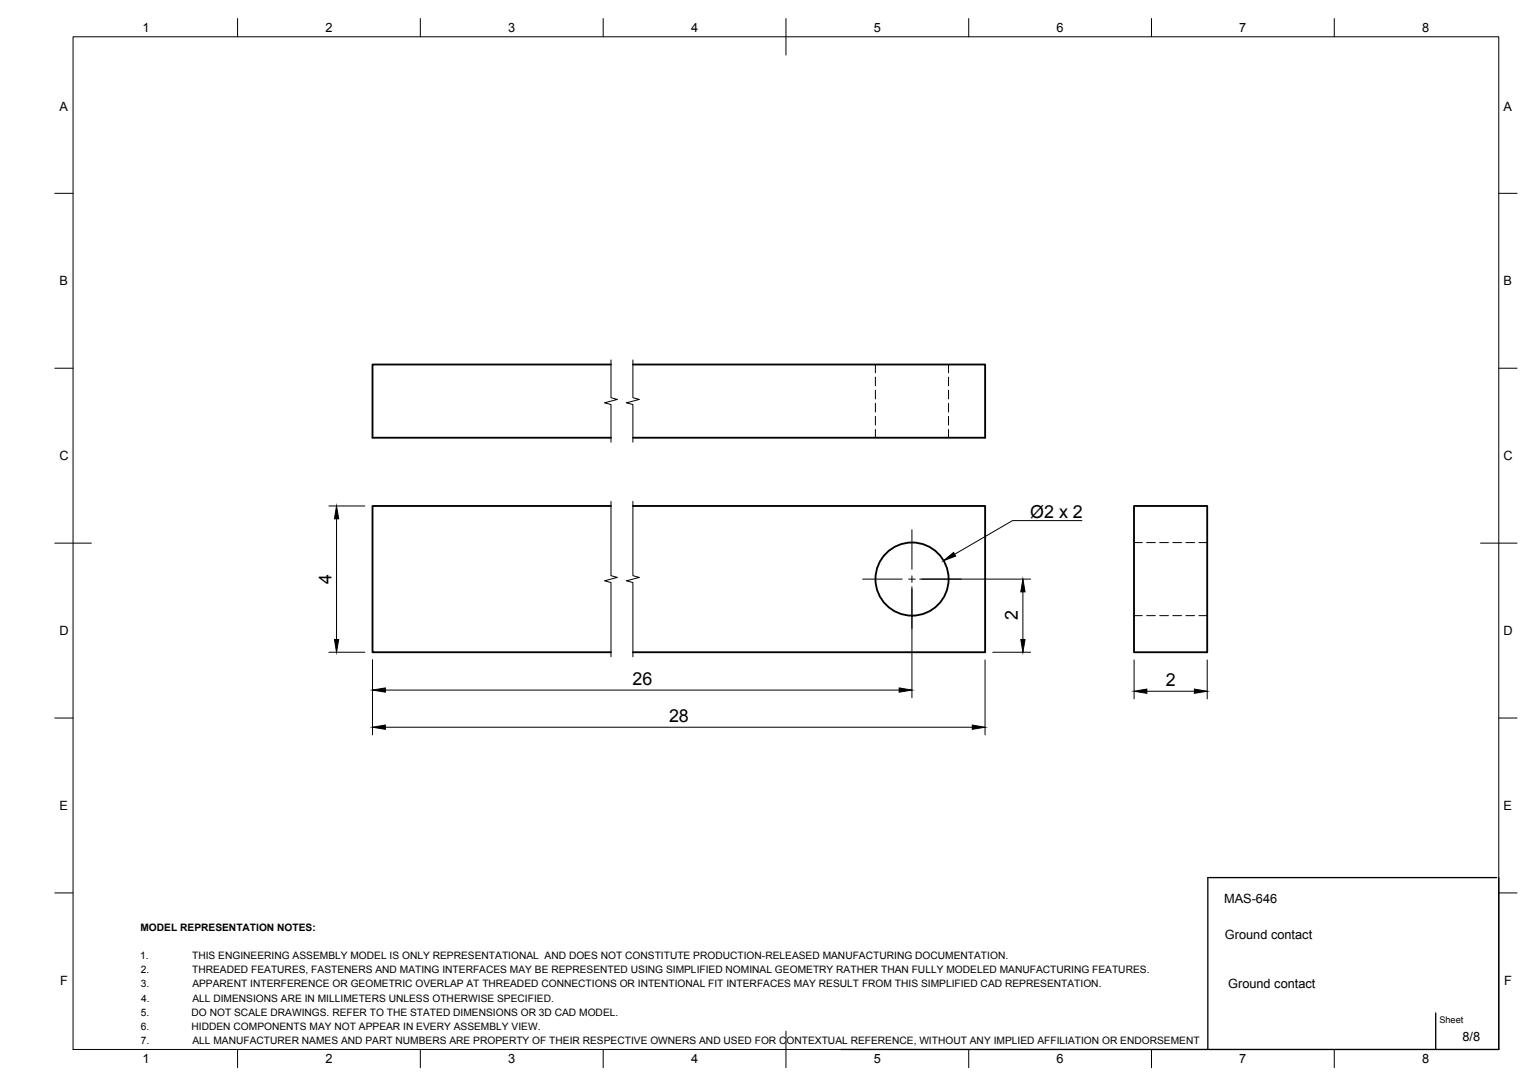
ISO-10303-21;
HEADER;
/* Generated by software containing ST-Developer
 * from STEP Tools, Inc. (www.steptools.com) 
 */

FILE_DESCRIPTION(
/* description */ ('Independent keyed three-contact power inlet for the IEC-connector des
ign category. Longer ground blade, retained contacts, wire termination
 holes and sealed bolted panel interface. Nominal custom interface; IE
C dimensional compatibility and electrical ratings are not assigned.'),

/* implementation_level */ '2;1');

FILE_NAME(
/* name */ 'Ground contact.step',
/* time_stamp */ '2026-11-08T19:55:04-08:00',
/* author */ (''),
/* organization */ (''),
/* preprocessor_version */ 'ST-DEVELOPER v20.2',
/* originating_system */ 'Autodesk Translation Framework v15.17.0.0',
/* authorisation */ '');

FILE_SCHEMA (('AUTOMOTIVE_DESIGN { 1 0 10303 214 3 1 1 }'));
ENDSEC;

DATA;
#10=MECHANICAL_DESIGN_GEOMETRIC_PRESENTATION_REPRESENTATION('',(#113),#21880);
#93=SHAPE_REPRESENTATION_RELATIONSHIP('SRR','None',#21929,#103);
#103=ADVANCED_BREP_SHAPE_REPRESENTATION('',(#123),#21874);
#113=STYLED_ITEM('',(#21988),#123);
#123=MANIFOLD_SOLID_BREP('Body1',#6385);
#185=FACE_BOUND('',#935,.T.);
#186=FACE_BOUND('',#938,.T.);
#271=PLANE('',#6806);
#272=PLANE('',#6807);
#273=PLANE('',#6808);
#274=PLANE('',#6809);
#275=PLANE('',#6810);
#276=PLANE('',#6811);
#547=FACE_OUTER_BOUND('',#933,.T.);
#548=FACE_OUTER_BOUND('',#934,.T.);
#549=FACE_OUTER_BOUND('',#936,.T.);
#550=FACE_OUTER_BOUND('',#937,.T.);
#551=FACE_OUTER_BOUND('',#939,.T.);
#552=FACE_OUTER_BOUND('',#940,.T.);
#553=FACE_OUTER_BOUND('',#941,.T.);
#933=EDGE_LOOP('',(#5195,#5196,#5197,#5198));
#934=EDGE_LOOP('',(#5199,#5200,#5201,#5202));
#935=EDGE_LOOP('',(#5203));
#936=EDGE_LOOP('',(#5204,#5205,#5206,#5207));
#937=EDGE_LOOP('',(#5208,#5209,#5210,#5211));
#938=EDGE_LOOP('',(#5212));
#939=EDGE_LOOP('',(#5213,#5214,#5215,#5216));
#940=EDGE_LOOP('',(#5217,#5218,#5219,#5220));
#941=EDGE_LOOP('',(#5221,#5222,#5223,#5224));
#1136=CIRCLE('',#6804,1.);
#1137=CIRCLE('',#6805,1.);
#1839=LINE('',#16286,#2295);
#1840=LINE('',#16291,#2296);
#1841=LINE('',#16293,#2297);
#1842=LINE('',#16295,#2298);
#1843=LINE('',#16296,#2299);
#1844=LINE('',#16299,#2300);
#1845=LINE('',#16301,#2301);
#1846=LINE('',#16302,#2302);
#1847=LINE('',#16305,#2303);
#1848=LINE('',#16307,#2304);
#1849=LINE('',#16308,#2305);
#1850=LINE('',#16310,#2306);
#1851=LINE('',#16311,#2307);
#2295=VECTOR('',#7883,1.);
#2296=VECTOR('',#7888,10.);
#2297=VECTOR('',#7889,10.);
#2298=VECTOR('',#7890,10.);
#2299=VECTOR('',#7891,10.);
#2300=VECTOR('',#7894,10.);
#2301=VECTOR('',#7895,10.);
#2302=VECTOR('',#7896,10.);
#2303=VECTOR('',#7899,10.);
#2304=VECTOR('',#7900,10.);
#2305=VECTOR('',#7901,10.);
#2306=VECTOR('',#7904,10.);
#2307=VECTOR('',#7905,10.);
#2835=VERTEX_POINT('',#16283);
#2836=VERTEX_POINT('',#16285);
#2837=VERTEX_POINT('',#16289);
#2838=VERTEX_POINT('',#16290);
#2839=VERTEX_POINT('',#16292);
#2840=VERTEX_POINT('',#16294);
#2841=VERTEX_POINT('',#16298);
#2842=VERTEX_POINT('',#16300);
#2843=VERTEX_POINT('',#16304);
#2844=VERTEX_POINT('',#16306);
#3657=EDGE_CURVE('',#2835,#2835,#1136,.T.);
#3658=EDGE_CURVE('',#2835,#2836,#1839,.T.);
#3659=EDGE_CURVE('',#2836,#2836,#1137,.T.);
#3660=EDGE_CURVE('',#2837,#2838,#1840,.T.);
#3661=EDGE_CURVE('',#2838,#2839,#1841,.T.);
#3662=EDGE_CURVE('',#2840,#2839,#1842,.T.);
#3663=EDGE_CURVE('',#2837,#2840,#1843,.T.);
#3664=EDGE_CURVE('',#2841,#2837,#1844,.T.);
#3665=EDGE_CURVE('',#2842,#2840,#1845,.T.);
#3666=EDGE_CURVE('',#2841,#2842,#1846,.T.);
#3667=EDGE_CURVE('',#2843,#2841,#1847,.T.);
#3668=EDGE_CURVE('',#2844,#2842,#1848,.T.);
#3669=EDGE_CURVE('',#2843,#2844,#1849,.T.);
#3670=EDGE_CURVE('',#2838,#2843,#1850,.T.);
#3671=EDGE_CURVE('',#2839,#2844,#1851,.T.);
#5195=ORIENTED_EDGE('',*,*,#3657,.F.);
#5196=ORIENTED_EDGE('',*,*,#3658,.T.);
#5197=ORIENTED_EDGE('',*,*,#3659,.F.);
#5198=ORIENTED_EDGE('',*,*,#3658,.F.);
#5199=ORIENTED_EDGE('',*,*,#3660,.T.);
#5200=ORIENTED_EDGE('',*,*,#3661,.T.);
#5201=ORIENTED_EDGE('',*,*,#3662,.F.);
#5202=ORIENTED_EDGE('',*,*,#3663,.F.);
#5203=ORIENTED_EDGE('',*,*,#3657,.T.);
#5204=ORIENTED_EDGE('',*,*,#3664,.T.);
#5205=ORIENTED_EDGE('',*,*,#3663,.T.);
#5206=ORIENTED_EDGE('',*,*,#3665,.F.);
#5207=ORIENTED_EDGE('',*,*,#3666,.F.);
#5208=ORIENTED_EDGE('',*,*,#3667,.T.);
#5209=ORIENTED_EDGE('',*,*,#3666,.T.);
#5210=ORIENTED_EDGE('',*,*,#3668,.F.);
#5211=ORIENTED_EDGE('',*,*,#3669,.F.);
#5212=ORIENTED_EDGE('',*,*,#3659,.T.);
#5213=ORIENTED_EDGE('',*,*,#3670,.T.);
#5214=ORIENTED_EDGE('',*,*,#3669,.T.);
#5215=ORIENTED_EDGE('',*,*,#3671,.F.);
#5216=ORIENTED_EDGE('',*,*,#3661,.F.);
#5217=ORIENTED_EDGE('',*,*,#3671,.T.);
#5218=ORIENTED_EDGE('',*,*,#3668,.T.);
#5219=ORIENTED_EDGE('',*,*,#3665,.T.);
#5220=ORIENTED_EDGE('',*,*,#3662,.T.);
#5221=ORIENTED_EDGE('',*,*,#3670,.F.);
#5222=ORIENTED_EDGE('',*,*,#3660,.F.);
#5223=ORIENTED_EDGE('',*,*,#3664,.F.);
#5224=ORIENTED_EDGE('',*,*,#3667,.F.);
#5963=CYLINDRICAL_SURFACE('',#6803,1.);
#6259=ADVANCED_FACE('',(#547),#5963,.F.);
#6260=ADVANCED_FACE('',(#548,#185),#271,.T.);
#6261=ADVANCED_FACE('',(#549),#272,.T.);
#6262=ADVANCED_FACE('',(#550,#186),#273,.T.);
#6263=ADVANCED_FACE('',(#551),#274,.T.);
#6264=ADVANCED_FACE('',(#552),#275,.T.);
#6265=ADVANCED_FACE('',(#553),#276,.F.);
#6385=CLOSED_SHELL('',(#6259,#6260,#6261,#6262,#6263,#6264,#6265));
#6802=AXIS2_PLACEMENT_3D('',#16281,#7877,#7878);
#6803=AXIS2_PLACEMENT_3D('',#16282,#7879,#7880);
#6804=AXIS2_PLACEMENT_3D('',#16284,#7881,#7882);
#6805=AXIS2_PLACEMENT_3D('',#16287,#7884,#7885);
#6806=AXIS2_PLACEMENT_3D('',#16288,#7886,#7887);
#6807=AXIS2_PLACEMENT_3D('',#16297,#7892,#7893);
#6808=AXIS2_PLACEMENT_3D('',#16303,#7897,#7898);
#6809=AXIS2_PLACEMENT_3D('',#16309,#7902,#7903);
#6810=AXIS2_PLACEMENT_3D('',#16312,#7906,#7907);
#6811=AXIS2_PLACEMENT_3D('',#16313,#7908,#7909);
#7877=DIRECTION('axis',(0.,0.,1.));
#7878=DIRECTION('refdir',(1.,0.,0.));
#7879=DIRECTION('center_axis',(0.,-1.,0.));
#7880=DIRECTION('ref_axis',(0.,0.,1.));
#7881=DIRECTION('center_axis',(0.,-1.,0.));
#7882=DIRECTION('ref_axis',(0.,0.,1.));
#7883=DIRECTION('',(0.,-1.,0.));
#7884=DIRECTION('center_axis',(0.,1.,0.));
#7885=DIRECTION('ref_axis',(0.,0.,1.));
#7886=DIRECTION('center_axis',(0.,1.,0.));
#7887=DIRECTION('ref_axis',(-1.,0.,0.));
#7888=DIRECTION('',(-1.,0.,0.));
#7889=DIRECTION('',(0.,0.,1.));
#7890=DIRECTION('',(-1.,0.,0.));
#7891=DIRECTION('',(0.,0.,1.));
#7892=DIRECTION('center_axis',(1.,0.,0.));
#7893=DIRECTION('ref_axis',(0.,1.,0.));
#7894=DIRECTION('',(0.,1.,0.));
#7895=DIRECTION('',(0.,1.,0.));
#7896=DIRECTION('',(0.,0.,1.));
#7897=DIRECTION('center_axis',(0.,-1.,0.));
#7898=DIRECTION('ref_axis',(1.,0.,0.));
#7899=DIRECTION('',(1.,0.,0.));
#7900=DIRECTION('',(1.,0.,0.));
#7901=DIRECTION('',(0.,0.,1.));
#7902=DIRECTION('center_axis',(-1.,0.,0.));
#7903=DIRECTION('ref_axis',(0.,-1.,0.));
#7904=DIRECTION('',(0.,-1.,0.));
#7905=DIRECTION('',(0.,-1.,0.));
#7906=DIRECTION('center_axis',(0.,0.,1.));
#7907=DIRECTION('ref_axis',(1.,0.,0.));
#7908=DIRECTION('center_axis',(0.,0.,1.));
#7909=DIRECTION('ref_axis',(1.,0.,0.));
#16281=CARTESIAN_POINT('',(0.,0.,0.));
#16282=CARTESIAN_POINT('Origin',(0.,0.,2.));
#16283=CARTESIAN_POINT('',(1.22464679914735E-16,1.,1.));
#16284=CARTESIAN_POINT('Origin',(0.,1.,2.));
#16285=CARTESIAN_POINT('',(1.22464679914735E-16,-1.,1.));
#16286=CARTESIAN_POINT('',(1.22464679914735E-16,0.,1.));
#16287=CARTESIAN_POINT('Origin',(0.,-1.,2.));
#16288=CARTESIAN_POINT('Origin',(2.,1.,0.));
#16289=CARTESIAN_POINT('',(2.,1.,0.));
#16290=CARTESIAN_POINT('',(-2.,1.,0.));
#16291=CARTESIAN_POINT('',(2.,1.,0.));
#16292=CARTESIAN_POINT('',(-2.,1.,28.));
#16293=CARTESIAN_POINT('',(-2.,1.,0.));
#16294=CARTESIAN_POINT('',(2.,1.,28.));
#16295=CARTESIAN_POINT('',(2.,1.,28.));
#16296=CARTESIAN_POINT('',(2.,1.,0.));
#16297=CARTESIAN_POINT('Origin',(2.,-1.,0.));
#16298=CARTESIAN_POINT('',(2.,-1.,0.));
#16299=CARTESIAN_POINT('',(2.,-1.,0.));
#16300=CARTESIAN_POINT('',(2.,-1.,28.));
#16301=CARTESIAN_POINT('',(2.,-1.,28.));
#16302=CARTESIAN_POINT('',(2.,-1.,0.));
#16303=CARTESIAN_POINT('Origin',(-2.,-1.,0.));
#16304=CARTESIAN_POINT('',(-2.,-1.,0.));
#16305=CARTESIAN_POINT('',(-2.,-1.,0.));
#16306=CARTESIAN_POINT('',(-2.,-1.,28.));
#16307=CARTESIAN_POINT('',(-2.,-1.,28.));
#16308=CARTESIAN_POINT('',(-2.,-1.,0.));
#16309=CARTESIAN_POINT('Origin',(-2.,1.,0.));
#16310=CARTESIAN_POINT('',(-2.,1.,0.));
#16311=CARTESIAN_POINT('',(-2.,1.,28.));
#16312=CARTESIAN_POINT('Origin',(0.,0.,28.));
#16313=CARTESIAN_POINT('Origin',(0.,0.,0.));
#21862=UNCERTAINTY_MEASURE_WITH_UNIT(LENGTH_MEASURE(0.01),#21881,
'DISTANCE_ACCURACY_VALUE',
'Maximum model space distance between geometric entities at asserted c
onnectivities');
#21868=UNCERTAINTY_MEASURE_WITH_UNIT(LENGTH_MEASURE(0.01),#21881,
'DISTANCE_ACCURACY_VALUE',
'Maximum model space distance between geometric entities at asserted c
onnectivities');
#21874=(
GEOMETRIC_REPRESENTATION_CONTEXT(3)
GLOBAL_UNCERTAINTY_ASSIGNED_CONTEXT((#21862))
GLOBAL_UNIT_ASSIGNED_CONTEXT((#21881,#21883,#21884))
REPRESENTATION_CONTEXT('','3D')
);
#21880=(
GEOMETRIC_REPRESENTATION_CONTEXT(3)
GLOBAL_UNCERTAINTY_ASSIGNED_CONTEXT((#21868))
GLOBAL_UNIT_ASSIGNED_CONTEXT((#21881,#21883,#21884))
REPRESENTATION_CONTEXT('','3D')
);
#21881=(
LENGTH_UNIT()
NAMED_UNIT(*)
SI_UNIT(.MILLI.,.METRE.)
);
#21883=(
NAMED_UNIT(*)
PLANE_ANGLE_UNIT()
SI_UNIT($,.RADIAN.)
);
#21884=(
NAMED_UNIT(*)
SI_UNIT($,.STERADIAN.)
SOLID_ANGLE_UNIT()
);
#21890=SHAPE_DEFINITION_REPRESENTATION(#21901,#21929);
#21901=PRODUCT_DEFINITION_SHAPE('',$,#21941);
#21929=SHAPE_REPRESENTATION('',(#6802),#21874);
#21935=PRODUCT_DEFINITION_CONTEXT('part definition',#21970,'design');
#21941=PRODUCT_DEFINITION('Ground contact','Ground contact',#21952,#21935);
#21952=PRODUCT_DEFINITION_FORMATION('',$,#21977);
#21970=APPLICATION_CONTEXT(
'Core Data for Automotive Mechanical Design Process');
#21971=PRODUCT_CONTEXT('part definition',#21970,'mechanical');
#21977=PRODUCT('Ground contact','Ground contact',$,(#21971));
#21988=PRESENTATION_STYLE_ASSIGNMENT((#21994));
#21994=SURFACE_STYLE_USAGE(.BOTH.,#22000);
#22000=SURFACE_SIDE_STYLE('',(#22006));
#22006=SURFACE_STYLE_FILL_AREA(#22012);
#22012=FILL_AREA_STYLE('Light gray',(#22018));
#22018=FILL_AREA_STYLE_COLOUR('Light gray',#22024);
#22024=COLOUR_RGB('Light gray',0.725490196078431,0.752941176470588,0.792156862745098);
ENDSEC;
END-ISO-10303-21;
